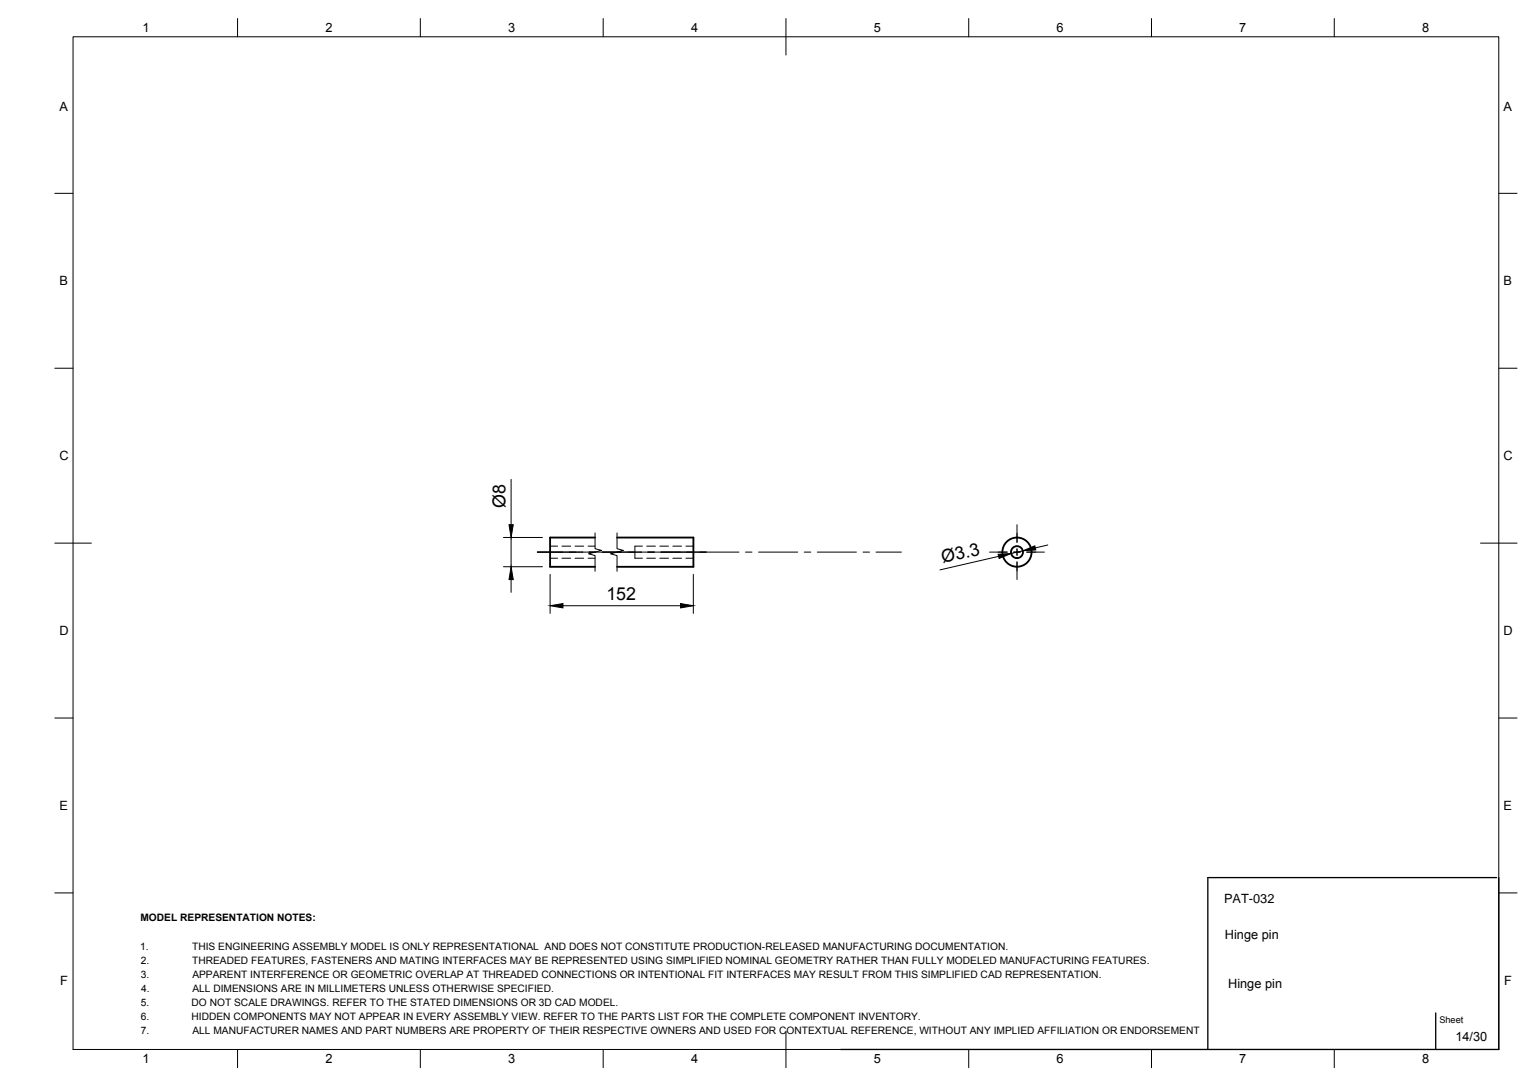
ISO-10303-21;
HEADER;
/* Generated by software containing ST-Developer
 * from STEP Tools, Inc. (www.steptools.com) 
 */

FILE_DESCRIPTION(
/* description */ ('Drill jig with bushing plate'),
/* implementation_level */ '2;1');

FILE_NAME(
/* name */ 'Hinge pin.step',
/* time_stamp */ '2026-10-27T10:51:08-07:00',
/* author */ (''),
/* organization */ (''),
/* preprocessor_version */ 'ST-DEVELOPER v20.2',
/* originating_system */ 'Autodesk Translation Framework v15.17.0.0',
/* authorisation */ '');

FILE_SCHEMA (('AUTOMOTIVE_DESIGN { 1 0 10303 214 3 1 1 }'));
ENDSEC;

DATA;
#10=MECHANICAL_DESIGN_GEOMETRIC_PRESENTATION_REPRESENTATION('',(#232),#6638);
#184=SHAPE_REPRESENTATION_RELATIONSHIP('SRR','None',#6748,#208);
#208=ADVANCED_BREP_SHAPE_REPRESENTATION('',(#256),#6621);
#232=STYLED_ITEM('',(#6943),#256);
#256=MANIFOLD_SOLID_BREP('Body1',#3599);
#328=FACE_BOUND('',#867,.T.);
#329=FACE_BOUND('',#869,.T.);
#423=PLANE('',#4051);
#424=PLANE('',#4055);
#425=PLANE('',#4059);
#426=PLANE('',#4060);
#588=FACE_OUTER_BOUND('',#861,.T.);
#589=FACE_OUTER_BOUND('',#862,.T.);
#590=FACE_OUTER_BOUND('',#863,.T.);
#591=FACE_OUTER_BOUND('',#864,.T.);
#592=FACE_OUTER_BOUND('',#865,.T.);
#593=FACE_OUTER_BOUND('',#866,.T.);
#594=FACE_OUTER_BOUND('',#868,.T.);
#861=EDGE_LOOP('',(#2813,#2814,#2815,#2816));
#862=EDGE_LOOP('',(#2817));
#863=EDGE_LOOP('',(#2818,#2819,#2820,#2821));
#864=EDGE_LOOP('',(#2822));
#865=EDGE_LOOP('',(#2823,#2824,#2825,#2826));
#866=EDGE_LOOP('',(#2827));
#867=EDGE_LOOP('',(#2828));
#868=EDGE_LOOP('',(#2829));
#869=EDGE_LOOP('',(#2830));
#1148=LINE('',#6001,#1409);
#1149=LINE('',#6008,#1410);
#1150=LINE('',#6015,#1411);
#1409=VECTOR('',#4785,0.165);
#1410=VECTOR('',#4794,0.165);
#1411=VECTOR('',#4803,0.4);
#1620=CIRCLE('',#4049,0.165);
#1621=CIRCLE('',#4050,0.165);
#1622=CIRCLE('',#4053,0.165);
#1623=CIRCLE('',#4054,0.165);
#1624=CIRCLE('',#4057,0.4);
#1625=CIRCLE('',#4058,0.4);
#1846=VERTEX_POINT('',#5998);
#1847=VERTEX_POINT('',#6000);
#1848=VERTEX_POINT('',#6005);
#1849=VERTEX_POINT('',#6007);
#1850=VERTEX_POINT('',#6012);
#1851=VERTEX_POINT('',#6014);
#2194=EDGE_CURVE('',#1846,#1846,#1620,.T.);
#2195=EDGE_CURVE('',#1846,#1847,#1148,.T.);
#2196=EDGE_CURVE('',#1847,#1847,#1621,.T.);
#2197=EDGE_CURVE('',#1848,#1848,#1622,.T.);
#2198=EDGE_CURVE('',#1848,#1849,#1149,.T.);
#2199=EDGE_CURVE('',#1849,#1849,#1623,.T.);
#2200=EDGE_CURVE('',#1850,#1850,#1624,.T.);
#2201=EDGE_CURVE('',#1850,#1851,#1150,.T.);
#2202=EDGE_CURVE('',#1851,#1851,#1625,.T.);
#2813=ORIENTED_EDGE('',*,*,#2194,.F.);
#2814=ORIENTED_EDGE('',*,*,#2195,.T.);
#2815=ORIENTED_EDGE('',*,*,#2196,.F.);
#2816=ORIENTED_EDGE('',*,*,#2195,.F.);
#2817=ORIENTED_EDGE('',*,*,#2194,.T.);
#2818=ORIENTED_EDGE('',*,*,#2197,.F.);
#2819=ORIENTED_EDGE('',*,*,#2198,.T.);
#2820=ORIENTED_EDGE('',*,*,#2199,.T.);
#2821=ORIENTED_EDGE('',*,*,#2198,.F.);
#2822=ORIENTED_EDGE('',*,*,#2199,.F.);
#2823=ORIENTED_EDGE('',*,*,#2200,.F.);
#2824=ORIENTED_EDGE('',*,*,#2201,.T.);
#2825=ORIENTED_EDGE('',*,*,#2202,.T.);
#2826=ORIENTED_EDGE('',*,*,#2201,.F.);
#2827=ORIENTED_EDGE('',*,*,#2200,.T.);
#2828=ORIENTED_EDGE('',*,*,#2196,.T.);
#2829=ORIENTED_EDGE('',*,*,#2202,.F.);
#2830=ORIENTED_EDGE('',*,*,#2197,.T.);
#3333=CYLINDRICAL_SURFACE('',#4048,0.165);
#3334=CYLINDRICAL_SURFACE('',#4052,0.165);
#3335=CYLINDRICAL_SURFACE('',#4056,0.4);
#3463=ADVANCED_FACE('',(#588),#3333,.F.);
#3464=ADVANCED_FACE('',(#589),#423,.T.);
#3465=ADVANCED_FACE('',(#590),#3334,.F.);
#3466=ADVANCED_FACE('',(#591),#424,.F.);
#3467=ADVANCED_FACE('',(#592),#3335,.T.);
#3468=ADVANCED_FACE('',(#593,#328),#425,.T.);
#3469=ADVANCED_FACE('',(#594,#329),#426,.F.);
#3599=CLOSED_SHELL('',(#3463,#3464,#3465,#3466,#3467,#3468,#3469));
#4047=AXIS2_PLACEMENT_3D('',#5996,#4779,#4780);
#4048=AXIS2_PLACEMENT_3D('',#5997,#4781,#4782);
#4049=AXIS2_PLACEMENT_3D('',#5999,#4783,#4784);
#4050=AXIS2_PLACEMENT_3D('',#6002,#4786,#4787);
#4051=AXIS2_PLACEMENT_3D('',#6003,#4788,#4789);
#4052=AXIS2_PLACEMENT_3D('',#6004,#4790,#4791);
#4053=AXIS2_PLACEMENT_3D('',#6006,#4792,#4793);
#4054=AXIS2_PLACEMENT_3D('',#6009,#4795,#4796);
#4055=AXIS2_PLACEMENT_3D('',#6010,#4797,#4798);
#4056=AXIS2_PLACEMENT_3D('',#6011,#4799,#4800);
#4057=AXIS2_PLACEMENT_3D('',#6013,#4801,#4802);
#4058=AXIS2_PLACEMENT_3D('',#6016,#4804,#4805);
#4059=AXIS2_PLACEMENT_3D('',#6017,#4806,#4807);
#4060=AXIS2_PLACEMENT_3D('',#6018,#4808,#4809);
#4779=DIRECTION('axis',(0.,0.,1.));
#4780=DIRECTION('refdir',(1.,0.,0.));
#4781=DIRECTION('center_axis',(1.,0.,0.));
#4782=DIRECTION('ref_axis',(0.,0.,-1.));
#4783=DIRECTION('center_axis',(1.,0.,0.));
#4784=DIRECTION('ref_axis',(0.,0.,-1.));
#4785=DIRECTION('',(1.,0.,0.));
#4786=DIRECTION('center_axis',(-1.,0.,0.));
#4787=DIRECTION('ref_axis',(0.,0.,-1.));
#4788=DIRECTION('center_axis',(1.,0.,0.));
#4789=DIRECTION('ref_axis',(0.,0.,-1.));
#4790=DIRECTION('center_axis',(1.,0.,0.));
#4791=DIRECTION('ref_axis',(0.,0.,-1.));
#4792=DIRECTION('center_axis',(1.,0.,0.));
#4793=DIRECTION('ref_axis',(0.,0.,-1.));
#4794=DIRECTION('',(1.,0.,0.));
#4795=DIRECTION('center_axis',(1.,0.,0.));
#4796=DIRECTION('ref_axis',(0.,0.,-1.));
#4797=DIRECTION('center_axis',(1.,0.,0.));
#4798=DIRECTION('ref_axis',(0.,0.,-1.));
#4799=DIRECTION('center_axis',(1.,0.,0.));
#4800=DIRECTION('ref_axis',(0.,0.,-1.));
#4801=DIRECTION('center_axis',(1.,0.,0.));
#4802=DIRECTION('ref_axis',(0.,0.,-1.));
#4803=DIRECTION('',(-1.,0.,0.));
#4804=DIRECTION('center_axis',(1.,0.,0.));
#4805=DIRECTION('ref_axis',(0.,0.,-1.));
#4806=DIRECTION('center_axis',(1.,0.,0.));
#4807=DIRECTION('ref_axis',(0.,0.,-1.));
#4808=DIRECTION('center_axis',(1.,0.,0.));
#4809=DIRECTION('ref_axis',(0.,0.,-1.));
#5996=CARTESIAN_POINT('',(0.,0.,0.));
#5997=CARTESIAN_POINT('Origin',(6.,-6.,3.5));
#5998=CARTESIAN_POINT('',(6.,-6.,3.665));
#5999=CARTESIAN_POINT('Origin',(6.,-6.,3.5));
#6000=CARTESIAN_POINT('',(7.6,-6.,3.665));
#6001=CARTESIAN_POINT('',(6.,-6.,3.665));
#6002=CARTESIAN_POINT('Origin',(7.6,-6.,3.5));
#6003=CARTESIAN_POINT('Origin',(6.,-6.,3.5));
#6004=CARTESIAN_POINT('Origin',(-7.7,-6.,3.5));
#6005=CARTESIAN_POINT('',(-7.6,-6.,3.665));
#6006=CARTESIAN_POINT('Origin',(-7.6,-6.,3.5));
#6007=CARTESIAN_POINT('',(-6.,-6.,3.665));
#6008=CARTESIAN_POINT('',(-7.7,-6.,3.665));
#6009=CARTESIAN_POINT('Origin',(-6.,-6.,3.5));
#6010=CARTESIAN_POINT('Origin',(-6.,-6.,3.5));
#6011=CARTESIAN_POINT('Origin',(-7.6,-6.,3.5));
#6012=CARTESIAN_POINT('',(7.6,-6.,3.9));
#6013=CARTESIAN_POINT('Origin',(7.6,-6.,3.5));
#6014=CARTESIAN_POINT('',(-7.6,-6.,3.9));
#6015=CARTESIAN_POINT('',(-7.6,-6.,3.9));
#6016=CARTESIAN_POINT('Origin',(-7.6,-6.,3.5));
#6017=CARTESIAN_POINT('Origin',(7.6,-6.,3.5));
#6018=CARTESIAN_POINT('Origin',(-7.6,-6.,3.5));
#6592=UNCERTAINTY_MEASURE_WITH_UNIT(LENGTH_MEASURE(0.001),#6639,
'DISTANCE_ACCURACY_VALUE',
'Maximum model space distance between geometric entities at asserted c
onnectivities');
#6609=UNCERTAINTY_MEASURE_WITH_UNIT(LENGTH_MEASURE(0.001),#6639,
'DISTANCE_ACCURACY_VALUE',
'Maximum model space distance between geometric entities at asserted c
onnectivities');
#6621=(
GEOMETRIC_REPRESENTATION_CONTEXT(3)
GLOBAL_UNCERTAINTY_ASSIGNED_CONTEXT((#6592))
GLOBAL_UNIT_ASSIGNED_CONTEXT((#6639,#6641,#6642))
REPRESENTATION_CONTEXT('','3D')
);
#6638=(
GEOMETRIC_REPRESENTATION_CONTEXT(3)
GLOBAL_UNCERTAINTY_ASSIGNED_CONTEXT((#6609))
GLOBAL_UNIT_ASSIGNED_CONTEXT((#6639,#6641,#6642))
REPRESENTATION_CONTEXT('','3D')
);
#6639=(
LENGTH_UNIT()
NAMED_UNIT(*)
SI_UNIT(.CENTI.,.METRE.)
);
#6641=(
NAMED_UNIT(*)
PLANE_ANGLE_UNIT()
SI_UNIT($,.RADIAN.)
);
#6642=(
NAMED_UNIT(*)
SI_UNIT($,.STERADIAN.)
SOLID_ANGLE_UNIT()
);
#6654=SHAPE_DEFINITION_REPRESENTATION(#6682,#6748);
#6682=PRODUCT_DEFINITION_SHAPE('',$,#6777);
#6748=SHAPE_REPRESENTATION('',(#4047),#6621);
#6765=PRODUCT_DEFINITION_CONTEXT('part definition',#6851,'design');
#6777=PRODUCT_DEFINITION('Hinge pin','Hinge pin',#6805,#6765);
#6805=PRODUCT_DEFINITION_FORMATION('',$,#6864);
#6851=APPLICATION_CONTEXT(
'Core Data for Automotive Mechanical Design Process');
#6852=PRODUCT_CONTEXT('part definition',#6851,'mechanical');
#6864=PRODUCT('Hinge pin','Hinge pin','Hinge pin',(#6852));
#6937=COLOUR_RGB('Grey',0.48,0.52,0.57);
#6938=FILL_AREA_STYLE_COLOUR('',#6937);
#6939=FILL_AREA_STYLE('',(#6938));
#6940=SURFACE_STYLE_FILL_AREA(#6939);
#6941=SURFACE_SIDE_STYLE('',(#6940));
#6942=SURFACE_STYLE_USAGE(.BOTH.,#6941);
#6943=PRESENTATION_STYLE_ASSIGNMENT((#6942));
ENDSEC;
END-ISO-10303-21;
